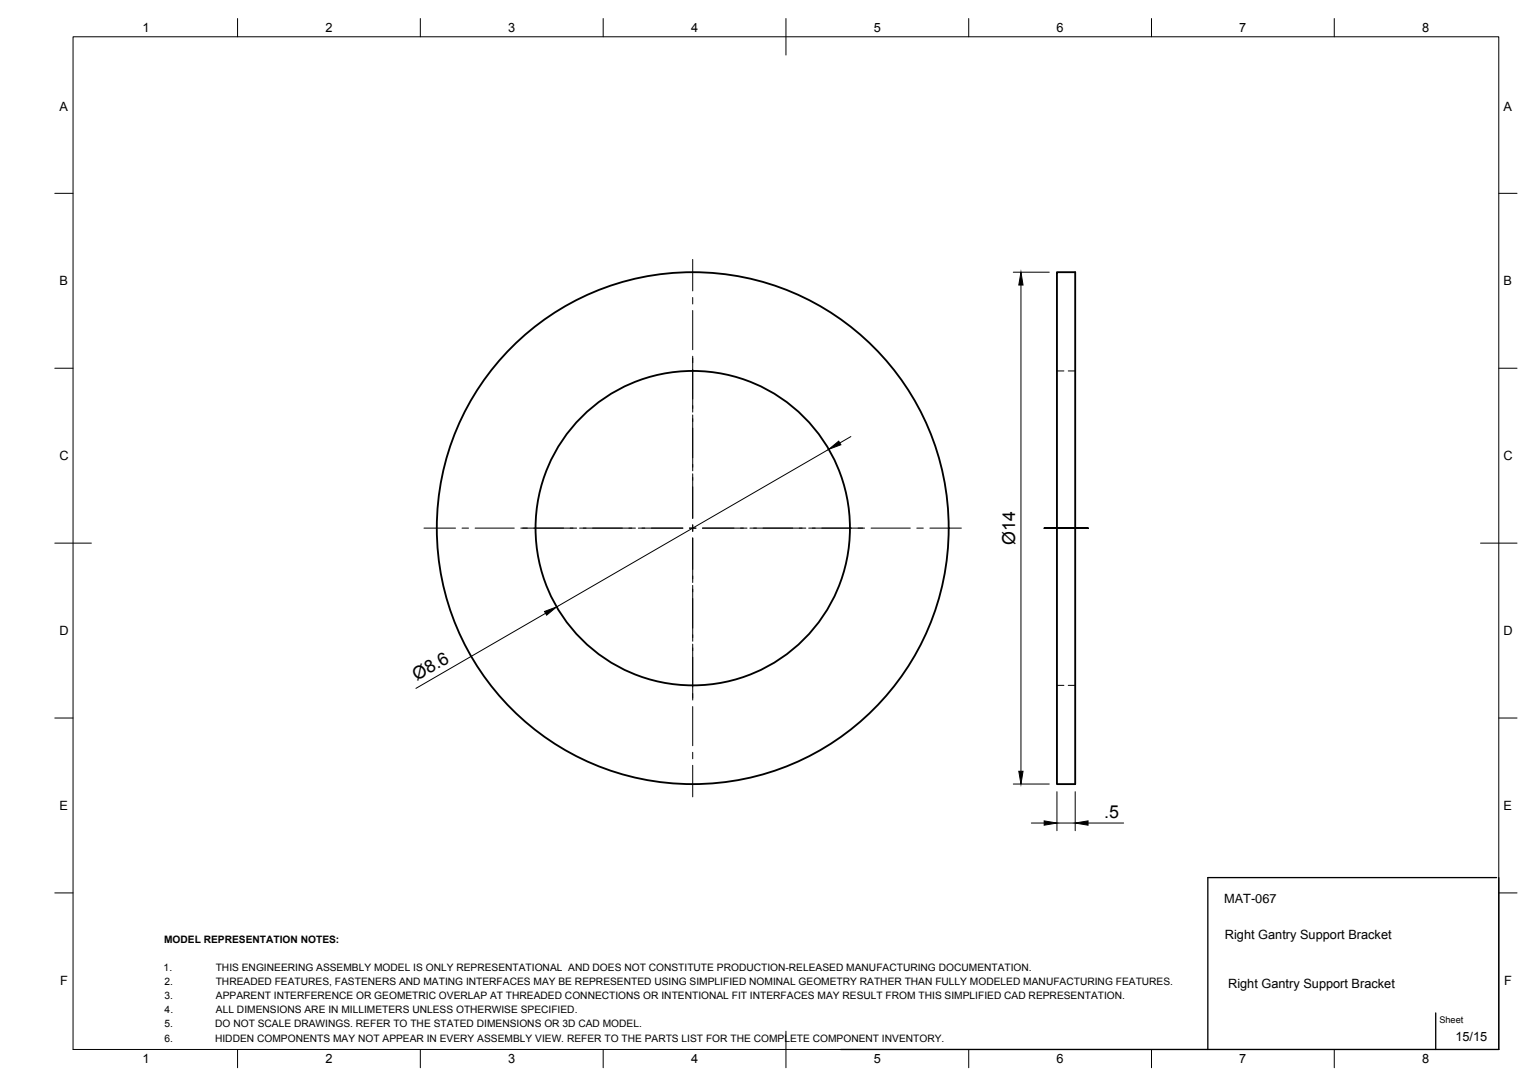
ISO-10303-21;
HEADER;
/* Generated by software containing ST-Developer
 * from STEP Tools, Inc. (www.steptools.com) 
 */

FILE_DESCRIPTION(
/* description */ ('CAx-IF Rec.Pracs.---Representation and Presentation of Product Manufa
cturing Information (PMI)---4.0---2014-10-13'),
/* implementation_level */ '2;1');

FILE_NAME(
/* name */ 'Right Gantry Support Bracket.step',
/* time_stamp */ '2026-10-24T16:02:03-07:00',
/* author */ (''),
/* organization */ (''),
/* preprocessor_version */ 'ST-DEVELOPER v20.2',
/* originating_system */ 'Autodesk Translation Framework v15.17.0.0',
/* authorisation */ '');

FILE_SCHEMA (('AP242_MANAGED_MODEL_BASED_3D_ENGINEERING_MIM_LF { 1 0 10303 442 2 1 4 }'));
ENDSEC;

DATA;
#10=MECHANICAL_DESIGN_GEOMETRIC_PRESENTATION_REPRESENTATION('',(#359),#6348);
#337=SHAPE_REPRESENTATION_RELATIONSHIP('SRR','None',#6499,#348);
#348=ADVANCED_BREP_SHAPE_REPRESENTATION('',(#370),#6347);
#359=STYLED_ITEM('',(#6603),#370);
#370=MANIFOLD_SOLID_BREP('Body1',#3398);
#462=CYLINDRICAL_SURFACE('',#3899,0.007);
#463=CYLINDRICAL_SURFACE('',#3903,0.0043);
#504=FACE_BOUND('',#1073,.T.);
#505=FACE_BOUND('',#1076,.T.);
#690=CIRCLE('',#3897,0.00700000000001);
#691=CIRCLE('',#3898,0.00430000000001);
#692=CIRCLE('',#3900,0.00700000000001);
#693=CIRCLE('',#3902,0.00430000000001);
#861=FACE_OUTER_BOUND('',#1072,.T.);
#862=FACE_OUTER_BOUND('',#1074,.T.);
#863=FACE_OUTER_BOUND('',#1075,.T.);
#864=FACE_OUTER_BOUND('',#1077,.T.);
#1072=EDGE_LOOP('',(#3125));
#1073=EDGE_LOOP('',(#3126));
#1074=EDGE_LOOP('',(#3127,#3128,#3129,#3130));
#1075=EDGE_LOOP('',(#3131));
#1076=EDGE_LOOP('',(#3132));
#1077=EDGE_LOOP('',(#3133,#3134,#3135,#3136));
#1309=LINE('',#6216,#1542);
#1310=LINE('',#6222,#1543);
#1542=VECTOR('',#4969,0.007);
#1543=VECTOR('',#4978,0.0043);
#1828=VERTEX_POINT('',#6210);
#1829=VERTEX_POINT('',#6212);
#1830=VERTEX_POINT('',#6215);
#1831=VERTEX_POINT('',#6219);
#2261=EDGE_CURVE('',#1828,#1828,#690,.T.);
#2262=EDGE_CURVE('',#1829,#1829,#691,.T.);
#2263=EDGE_CURVE('',#1828,#1830,#1309,.T.);
#2264=EDGE_CURVE('',#1830,#1830,#692,.T.);
#2265=EDGE_CURVE('',#1831,#1831,#693,.T.);
#2266=EDGE_CURVE('',#1831,#1829,#1310,.T.);
#3125=ORIENTED_EDGE('',*,*,#2261,.T.);
#3126=ORIENTED_EDGE('',*,*,#2262,.F.);
#3127=ORIENTED_EDGE('',*,*,#2261,.F.);
#3128=ORIENTED_EDGE('',*,*,#2263,.T.);
#3129=ORIENTED_EDGE('',*,*,#2264,.T.);
#3130=ORIENTED_EDGE('',*,*,#2263,.F.);
#3131=ORIENTED_EDGE('',*,*,#2264,.F.);
#3132=ORIENTED_EDGE('',*,*,#2265,.T.);
#3133=ORIENTED_EDGE('',*,*,#2265,.F.);
#3134=ORIENTED_EDGE('',*,*,#2266,.T.);
#3135=ORIENTED_EDGE('',*,*,#2262,.T.);
#3136=ORIENTED_EDGE('',*,*,#2266,.F.);
#3215=PLANE('',#3896);
#3216=PLANE('',#3901);
#3384=ADVANCED_FACE('',(#861,#504),#3215,.F.);
#3385=ADVANCED_FACE('',(#862),#462,.T.);
#3386=ADVANCED_FACE('',(#863,#505),#3216,.F.);
#3387=ADVANCED_FACE('',(#864),#463,.F.);
#3398=CLOSED_SHELL('',(#3384,#3385,#3386,#3387));
#3895=AXIS2_PLACEMENT_3D('',#6208,#4959,#4960);
#3896=AXIS2_PLACEMENT_3D('',#6209,#4961,#4962);
#3897=AXIS2_PLACEMENT_3D('',#6211,#4963,#4964);
#3898=AXIS2_PLACEMENT_3D('',#6213,#4965,#4966);
#3899=AXIS2_PLACEMENT_3D('',#6214,#4967,#4968);
#3900=AXIS2_PLACEMENT_3D('',#6217,#4970,#4971);
#3901=AXIS2_PLACEMENT_3D('',#6218,#4972,#4973);
#3902=AXIS2_PLACEMENT_3D('',#6220,#4974,#4975);
#3903=AXIS2_PLACEMENT_3D('',#6221,#4976,#4977);
#4959=DIRECTION('axis',(0.,0.,1.));
#4960=DIRECTION('refdir',(1.,0.,0.));
#4961=DIRECTION('center_axis',(0.,-1.,0.));
#4962=DIRECTION('ref_axis',(1.,0.,0.));
#4963=DIRECTION('center_axis',(0.,1.,0.));
#4964=DIRECTION('ref_axis',(1.,0.,0.));
#4965=DIRECTION('center_axis',(0.,1.,0.));
#4966=DIRECTION('ref_axis',(1.,0.,0.));
#4967=DIRECTION('center_axis',(0.,1.,0.));
#4968=DIRECTION('ref_axis',(0.,0.,1.));
#4969=DIRECTION('',(0.,-1.,0.));
#4970=DIRECTION('center_axis',(0.,1.,0.));
#4971=DIRECTION('ref_axis',(1.,0.,0.));
#4972=DIRECTION('center_axis',(0.,1.,0.));
#4973=DIRECTION('ref_axis',(0.,0.,1.));
#4974=DIRECTION('center_axis',(0.,1.,0.));
#4975=DIRECTION('ref_axis',(1.,0.,0.));
#4976=DIRECTION('center_axis',(0.,1.,0.));
#4977=DIRECTION('ref_axis',(0.,0.,1.));
#4978=DIRECTION('',(0.,1.,0.));
#6208=CARTESIAN_POINT('',(0.,0.,0.));
#6209=CARTESIAN_POINT('Origin',(0.,0.0109999997541308,0.00699999995096662));
#6210=CARTESIAN_POINT('',(-8.57252759403147E-19,0.0109999997541408,-0.00700000004903339));
#6211=CARTESIAN_POINT('Origin',(0.,0.0109999997541408,-4.90433850849834E-11));
#6212=CARTESIAN_POINT('',(-5.26598123633362E-19,0.0109999997541408,-0.00430000004903338));
#6213=CARTESIAN_POINT('Origin',(0.,0.0109999997541408,-4.90433850849834E-11));
#6214=CARTESIAN_POINT('Origin',(0.,0.0107499997597188,-4.90333850849834E-11));
#6215=CARTESIAN_POINT('',(-8.57252759403147E-19,0.0104999997653167,-0.00700000004903339));
#6216=CARTESIAN_POINT('',(-8.57252759403147E-19,0.0107499997597188,-0.00700000004903339));
#6217=CARTESIAN_POINT('Origin',(0.,0.0104999997653167,-4.90433850849834E-11));
#6218=CARTESIAN_POINT('Origin',(0.,0.0104999997653067,0.00429999995096661));
#6219=CARTESIAN_POINT('',(-5.26598123633362E-19,0.0104999997653167,-0.00430000004903338));
#6220=CARTESIAN_POINT('Origin',(0.,0.0104999997653167,-4.90433850849834E-11));
#6221=CARTESIAN_POINT('Origin',(0.,0.0107499997597188,-4.90333850849834E-11));
#6222=CARTESIAN_POINT('',(-5.26598123633362E-19,0.0107499997597188,-0.00430000004903338));
#6322=UNCERTAINTY_MEASURE_WITH_UNIT(LENGTH_MEASURE(1.E-5),#6349,
'DISTANCE_ACCURACY_VALUE',
'Maximum model space distance between geometric entities at asserted c
onnectivities');
#6323=UNCERTAINTY_MEASURE_WITH_UNIT(LENGTH_MEASURE(1.E-5),#6349,
'DISTANCE_ACCURACY_VALUE',
'Maximum model space distance between geometric entities at asserted c
onnectivities');
#6347=(
GEOMETRIC_REPRESENTATION_CONTEXT(3)
GLOBAL_UNCERTAINTY_ASSIGNED_CONTEXT((#6322))
GLOBAL_UNIT_ASSIGNED_CONTEXT((#6349,#6350,#6351))
REPRESENTATION_CONTEXT('','3D')
);
#6348=(
GEOMETRIC_REPRESENTATION_CONTEXT(3)
GLOBAL_UNCERTAINTY_ASSIGNED_CONTEXT((#6323))
GLOBAL_UNIT_ASSIGNED_CONTEXT((#6349,#6350,#6351))
REPRESENTATION_CONTEXT('','3D')
);
#6349=(
LENGTH_UNIT()
NAMED_UNIT(*)
SI_UNIT($,.METRE.)
);
#6350=(
NAMED_UNIT(*)
PLANE_ANGLE_UNIT()
SI_UNIT($,.RADIAN.)
);
#6351=(
NAMED_UNIT(*)
SI_UNIT($,.STERADIAN.)
SOLID_ANGLE_UNIT()
);
#6375=SHAPE_DEFINITION_REPRESENTATION(#6399,#6499);
#6399=PRODUCT_DEFINITION_SHAPE('',$,#6524);
#6499=SHAPE_REPRESENTATION('',(#3895),#6347);
#6500=PRODUCT_DEFINITION_CONTEXT('part definition',#6574,'design');
#6524=PRODUCT_DEFINITION('Right Gantry Support Bracket',
'Right Gantry Support Bracket',#6548,#6500);
#6548=PRODUCT_DEFINITION_FORMATION('',$,#6599);
#6574=APPLICATION_CONTEXT('Managed model based 3d engineering');
#6575=PRODUCT_CONTEXT('part definition',#6574,'mechanical');
#6599=PRODUCT('Right Gantry Support Bracket',
'Right Gantry Support Bracket',
'LEGAL AND USAGE DISCLAIMER: this Data/Model is provided \X2\201C\X0\A
S IS\X2\201D\X0\ for informational and representational only. It is a 
geometric approximation and is NOT engineered, certified, or guarantee
d for dimensional accuracy, exact tolerances, or production-level prec
ision. Vendor disclaims all implied warranties including fitness for a
 particular purpose. DO NOT USE FOR DIRECT PHYSICAL MANUFACTURING, AUT
OMATED PRODUCTION, OR SAFETY-CRITICAL SYSTEMS without independent engi
neering verification and resolution of any design discrepancies.',(#6575));
#6603=PRESENTATION_STYLE_ASSIGNMENT((#6609));
#6609=SURFACE_STYLE_USAGE(.BOTH.,#6615);
#6615=SURFACE_SIDE_STYLE('',(#6621));
#6621=SURFACE_STYLE_FILL_AREA(#6627);
#6627=FILL_AREA_STYLE('Opaque(137,137,137)',(#6633));
#6633=FILL_AREA_STYLE_COLOUR('Opaque(137,137,137)',#6639);
#6639=COLOUR_RGB('Opaque(137,137,137)',0.537254901960784,0.537254901960784,
0.537254901960784);
ENDSEC;
END-ISO-10303-21;
